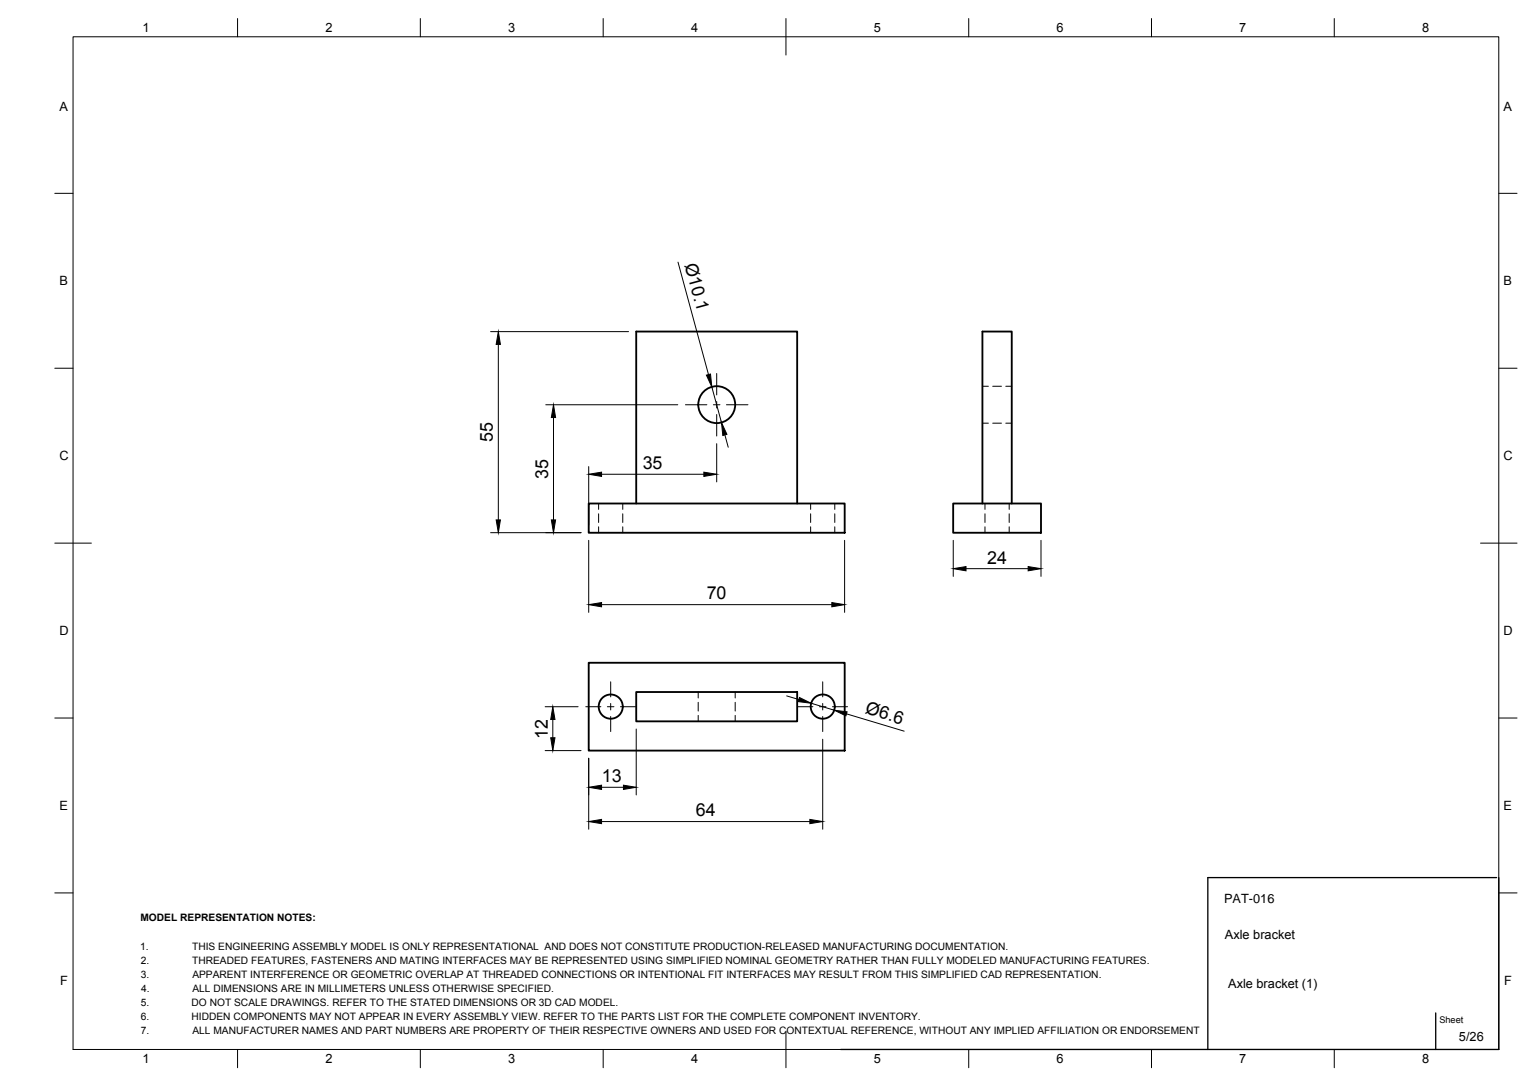
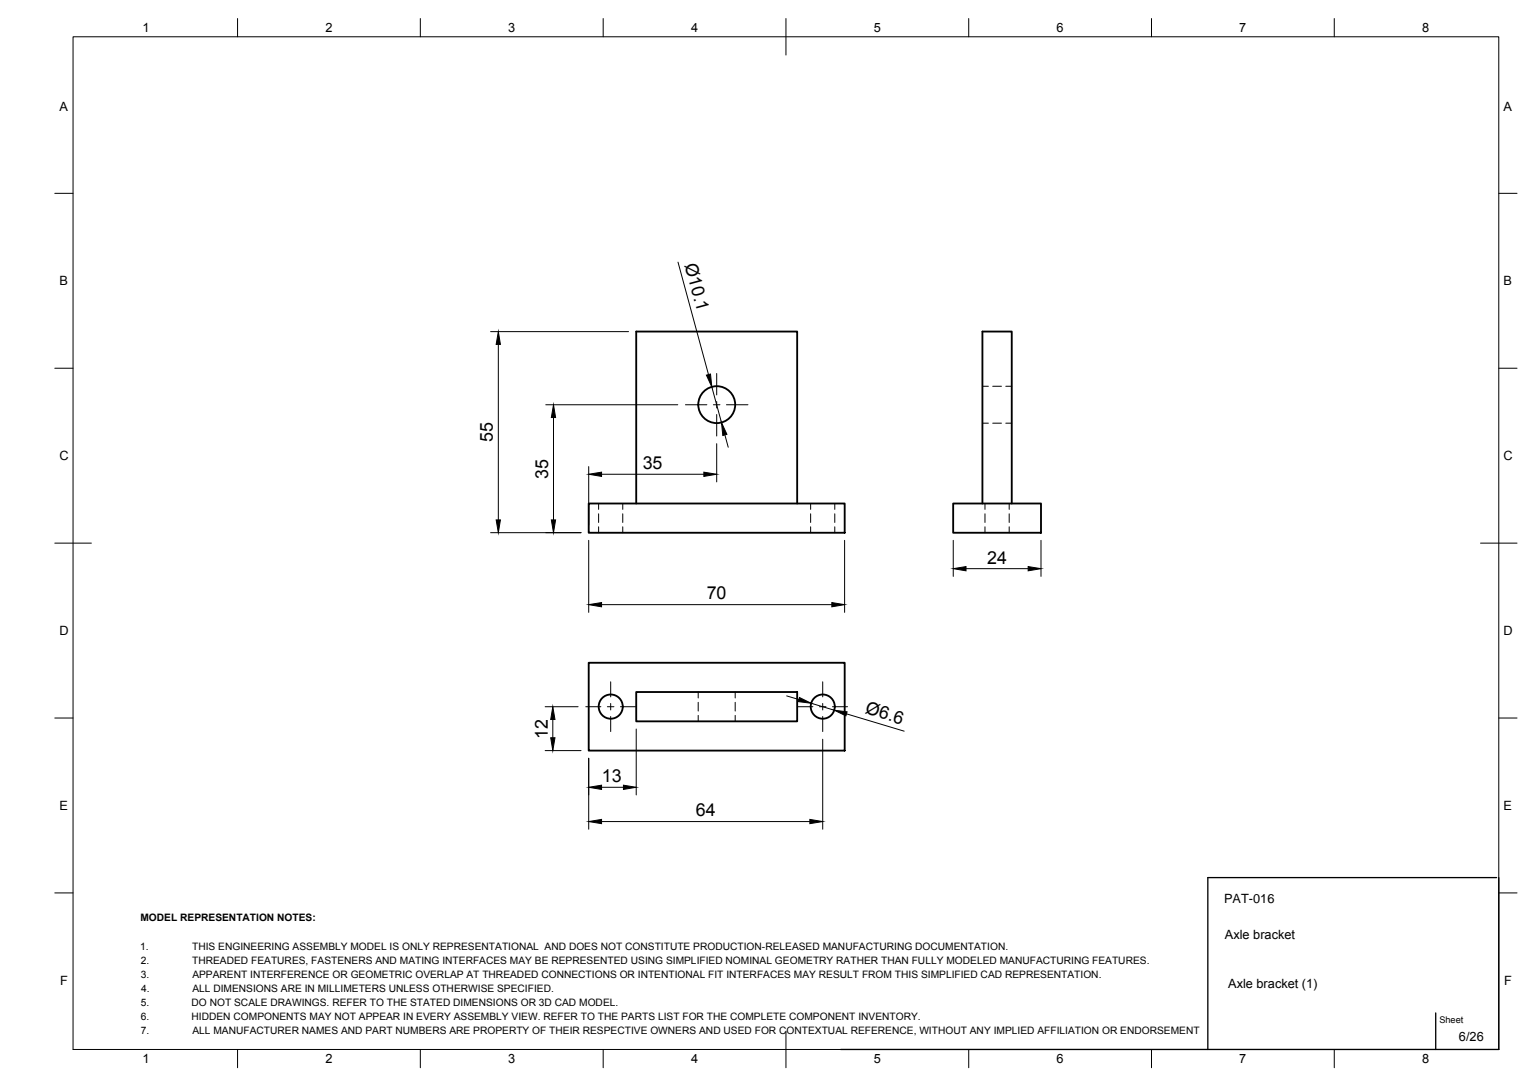
ISO-10303-21;
HEADER;
/* Generated by software containing ST-Developer
 * from STEP Tools, Inc. (www.steptools.com) 
 */

FILE_DESCRIPTION(
/* description */ ('Bracket-mounted idler roller'),
/* implementation_level */ '2;1');

FILE_NAME(
/* name */ 'Axle bracket.step',
/* time_stamp */ '2026-10-28T03:26:42-07:00',
/* author */ (''),
/* organization */ (''),
/* preprocessor_version */ 'ST-DEVELOPER v20.2',
/* originating_system */ 'Autodesk Translation Framework v15.17.0.0',
/* authorisation */ '');

FILE_SCHEMA (('AUTOMOTIVE_DESIGN { 1 0 10303 214 3 1 1 }'));
ENDSEC;

DATA;
#10=MECHANICAL_DESIGN_GEOMETRIC_PRESENTATION_REPRESENTATION('',(#280),#6241);
#238=SHAPE_REPRESENTATION_RELATIONSHIP('SRR','None',#6342,#259);
#259=ADVANCED_BREP_SHAPE_REPRESENTATION('',(#309),#6218);
#280=STYLED_ITEM('',(#6538),#309);
#309=MANIFOLD_SOLID_BREP('Body1',#3182);
#336=FACE_BOUND('',#711,.T.);
#337=FACE_BOUND('',#712,.T.);
#338=FACE_BOUND('',#713,.T.);
#339=FACE_BOUND('',#719,.T.);
#340=FACE_BOUND('',#722,.T.);
#341=FACE_BOUND('',#726,.T.);
#342=FACE_BOUND('',#727,.T.);
#417=PLANE('',#3457);
#418=PLANE('',#3458);
#419=PLANE('',#3459);
#420=PLANE('',#3460);
#421=PLANE('',#3461);
#422=PLANE('',#3462);
#423=PLANE('',#3463);
#424=PLANE('',#3464);
#425=PLANE('',#3465);
#426=PLANE('',#3466);
#427=PLANE('',#3467);
#516=FACE_OUTER_BOUND('',#707,.T.);
#517=FACE_OUTER_BOUND('',#708,.T.);
#518=FACE_OUTER_BOUND('',#709,.T.);
#519=FACE_OUTER_BOUND('',#710,.T.);
#520=FACE_OUTER_BOUND('',#714,.T.);
#521=FACE_OUTER_BOUND('',#715,.T.);
#522=FACE_OUTER_BOUND('',#716,.T.);
#523=FACE_OUTER_BOUND('',#717,.T.);
#524=FACE_OUTER_BOUND('',#718,.T.);
#525=FACE_OUTER_BOUND('',#720,.T.);
#526=FACE_OUTER_BOUND('',#721,.T.);
#527=FACE_OUTER_BOUND('',#723,.T.);
#528=FACE_OUTER_BOUND('',#724,.T.);
#529=FACE_OUTER_BOUND('',#725,.T.);
#707=EDGE_LOOP('',(#2166,#2167,#2168,#2169));
#708=EDGE_LOOP('',(#2170,#2171,#2172,#2173));
#709=EDGE_LOOP('',(#2174,#2175,#2176,#2177));
#710=EDGE_LOOP('',(#2178,#2179,#2180,#2181));
#711=EDGE_LOOP('',(#2182));
#712=EDGE_LOOP('',(#2183));
#713=EDGE_LOOP('',(#2184,#2185,#2186,#2187));
#714=EDGE_LOOP('',(#2188,#2189,#2190,#2191));
#715=EDGE_LOOP('',(#2192,#2193,#2194,#2195));
#716=EDGE_LOOP('',(#2196,#2197,#2198,#2199));
#717=EDGE_LOOP('',(#2200,#2201,#2202,#2203));
#718=EDGE_LOOP('',(#2204,#2205,#2206,#2207));
#719=EDGE_LOOP('',(#2208));
#720=EDGE_LOOP('',(#2209,#2210,#2211,#2212));
#721=EDGE_LOOP('',(#2213,#2214,#2215,#2216));
#722=EDGE_LOOP('',(#2217));
#723=EDGE_LOOP('',(#2218,#2219,#2220,#2221));
#724=EDGE_LOOP('',(#2222,#2223,#2224,#2225));
#725=EDGE_LOOP('',(#2226,#2227,#2228,#2229));
#726=EDGE_LOOP('',(#2230));
#727=EDGE_LOOP('',(#2231));
#979=LINE('',#4957,#1161);
#980=LINE('',#4963,#1162);
#981=LINE('',#4969,#1163);
#982=LINE('',#4974,#1164);
#983=LINE('',#4976,#1165);
#984=LINE('',#4978,#1166);
#985=LINE('',#4979,#1167);
#986=LINE('',#4982,#1168);
#987=LINE('',#4984,#1169);
#988=LINE('',#4986,#1170);
#989=LINE('',#4987,#1171);
#990=LINE('',#4990,#1172);
#991=LINE('',#4992,#1173);
#992=LINE('',#4993,#1174);
#993=LINE('',#4996,#1175);
#994=LINE('',#4998,#1176);
#995=LINE('',#4999,#1177);
#996=LINE('',#5001,#1178);
#997=LINE('',#5003,#1179);
#998=LINE('',#5006,#1180);
#999=LINE('',#5008,#1181);
#1000=LINE('',#5009,#1182);
#1001=LINE('',#5012,#1183);
#1002=LINE('',#5013,#1184);
#1003=LINE('',#5016,#1185);
#1004=LINE('',#5017,#1186);
#1005=LINE('',#5019,#1187);
#1161=VECTOR('',#3896,0.33);
#1162=VECTOR('',#3903,0.33);
#1163=VECTOR('',#3910,0.505);
#1164=VECTOR('',#3915,1.);
#1165=VECTOR('',#3916,1.);
#1166=VECTOR('',#3917,1.);
#1167=VECTOR('',#3918,1.);
#1168=VECTOR('',#3919,1.);
#1169=VECTOR('',#3920,1.);
#1170=VECTOR('',#3921,1.);
#1171=VECTOR('',#3922,1.);
#1172=VECTOR('',#3925,1.);
#1173=VECTOR('',#3926,1.);
#1174=VECTOR('',#3927,1.);
#1175=VECTOR('',#3930,1.);
#1176=VECTOR('',#3931,1.);
#1177=VECTOR('',#3932,1.);
#1178=VECTOR('',#3935,1.);
#1179=VECTOR('',#3938,1.);
#1180=VECTOR('',#3941,1.);
#1181=VECTOR('',#3942,1.);
#1182=VECTOR('',#3943,1.);
#1183=VECTOR('',#3946,1.);
#1184=VECTOR('',#3947,1.);
#1185=VECTOR('',#3950,1.);
#1186=VECTOR('',#3951,1.);
#1187=VECTOR('',#3954,1.);
#1343=CIRCLE('',#3449,0.33);
#1344=CIRCLE('',#3450,0.33);
#1345=CIRCLE('',#3452,0.33);
#1346=CIRCLE('',#3453,0.33);
#1347=CIRCLE('',#3455,0.505);
#1348=CIRCLE('',#3456,0.505);
#1524=VERTEX_POINT('',#4954);
#1525=VERTEX_POINT('',#4956);
#1526=VERTEX_POINT('',#4960);
#1527=VERTEX_POINT('',#4962);
#1528=VERTEX_POINT('',#4966);
#1529=VERTEX_POINT('',#4968);
#1530=VERTEX_POINT('',#4972);
#1531=VERTEX_POINT('',#4973);
#1532=VERTEX_POINT('',#4975);
#1533=VERTEX_POINT('',#4977);
#1534=VERTEX_POINT('',#4980);
#1535=VERTEX_POINT('',#4981);
#1536=VERTEX_POINT('',#4983);
#1537=VERTEX_POINT('',#4985);
#1538=VERTEX_POINT('',#4989);
#1539=VERTEX_POINT('',#4991);
#1540=VERTEX_POINT('',#4995);
#1541=VERTEX_POINT('',#4997);
#1542=VERTEX_POINT('',#5005);
#1543=VERTEX_POINT('',#5007);
#1544=VERTEX_POINT('',#5011);
#1545=VERTEX_POINT('',#5015);
#1785=EDGE_CURVE('',#1524,#1524,#1343,.T.);
#1786=EDGE_CURVE('',#1524,#1525,#979,.T.);
#1787=EDGE_CURVE('',#1525,#1525,#1344,.T.);
#1788=EDGE_CURVE('',#1526,#1526,#1345,.T.);
#1789=EDGE_CURVE('',#1526,#1527,#980,.T.);
#1790=EDGE_CURVE('',#1527,#1527,#1346,.T.);
#1791=EDGE_CURVE('',#1528,#1528,#1347,.T.);
#1792=EDGE_CURVE('',#1528,#1529,#981,.T.);
#1793=EDGE_CURVE('',#1529,#1529,#1348,.T.);
#1794=EDGE_CURVE('',#1530,#1531,#982,.T.);
#1795=EDGE_CURVE('',#1530,#1532,#983,.T.);
#1796=EDGE_CURVE('',#1533,#1532,#984,.T.);
#1797=EDGE_CURVE('',#1531,#1533,#985,.T.);
#1798=EDGE_CURVE('',#1534,#1535,#986,.T.);
#1799=EDGE_CURVE('',#1536,#1534,#987,.T.);
#1800=EDGE_CURVE('',#1537,#1536,#988,.T.);
#1801=EDGE_CURVE('',#1535,#1537,#989,.T.);
#1802=EDGE_CURVE('',#1531,#1538,#990,.T.);
#1803=EDGE_CURVE('',#1539,#1533,#991,.T.);
#1804=EDGE_CURVE('',#1538,#1539,#992,.T.);
#1805=EDGE_CURVE('',#1540,#1530,#993,.T.);
#1806=EDGE_CURVE('',#1540,#1541,#994,.T.);
#1807=EDGE_CURVE('',#1532,#1541,#995,.T.);
#1808=EDGE_CURVE('',#1541,#1539,#996,.T.);
#1809=EDGE_CURVE('',#1538,#1540,#997,.T.);
#1810=EDGE_CURVE('',#1536,#1542,#998,.T.);
#1811=EDGE_CURVE('',#1543,#1542,#999,.T.);
#1812=EDGE_CURVE('',#1537,#1543,#1000,.T.);
#1813=EDGE_CURVE('',#1534,#1544,#1001,.T.);
#1814=EDGE_CURVE('',#1542,#1544,#1002,.T.);
#1815=EDGE_CURVE('',#1535,#1545,#1003,.T.);
#1816=EDGE_CURVE('',#1544,#1545,#1004,.T.);
#1817=EDGE_CURVE('',#1545,#1543,#1005,.T.);
#2166=ORIENTED_EDGE('',*,*,#1785,.F.);
#2167=ORIENTED_EDGE('',*,*,#1786,.T.);
#2168=ORIENTED_EDGE('',*,*,#1787,.F.);
#2169=ORIENTED_EDGE('',*,*,#1786,.F.);
#2170=ORIENTED_EDGE('',*,*,#1788,.F.);
#2171=ORIENTED_EDGE('',*,*,#1789,.T.);
#2172=ORIENTED_EDGE('',*,*,#1790,.F.);
#2173=ORIENTED_EDGE('',*,*,#1789,.F.);
#2174=ORIENTED_EDGE('',*,*,#1791,.F.);
#2175=ORIENTED_EDGE('',*,*,#1792,.T.);
#2176=ORIENTED_EDGE('',*,*,#1793,.F.);
#2177=ORIENTED_EDGE('',*,*,#1792,.F.);
#2178=ORIENTED_EDGE('',*,*,#1794,.F.);
#2179=ORIENTED_EDGE('',*,*,#1795,.T.);
#2180=ORIENTED_EDGE('',*,*,#1796,.F.);
#2181=ORIENTED_EDGE('',*,*,#1797,.F.);
#2182=ORIENTED_EDGE('',*,*,#1787,.T.);
#2183=ORIENTED_EDGE('',*,*,#1790,.T.);
#2184=ORIENTED_EDGE('',*,*,#1798,.F.);
#2185=ORIENTED_EDGE('',*,*,#1799,.F.);
#2186=ORIENTED_EDGE('',*,*,#1800,.F.);
#2187=ORIENTED_EDGE('',*,*,#1801,.F.);
#2188=ORIENTED_EDGE('',*,*,#1802,.F.);
#2189=ORIENTED_EDGE('',*,*,#1797,.T.);
#2190=ORIENTED_EDGE('',*,*,#1803,.F.);
#2191=ORIENTED_EDGE('',*,*,#1804,.F.);
#2192=ORIENTED_EDGE('',*,*,#1805,.F.);
#2193=ORIENTED_EDGE('',*,*,#1806,.T.);
#2194=ORIENTED_EDGE('',*,*,#1807,.F.);
#2195=ORIENTED_EDGE('',*,*,#1795,.F.);
#2196=ORIENTED_EDGE('',*,*,#1796,.T.);
#2197=ORIENTED_EDGE('',*,*,#1807,.T.);
#2198=ORIENTED_EDGE('',*,*,#1808,.T.);
#2199=ORIENTED_EDGE('',*,*,#1803,.T.);
#2200=ORIENTED_EDGE('',*,*,#1794,.T.);
#2201=ORIENTED_EDGE('',*,*,#1802,.T.);
#2202=ORIENTED_EDGE('',*,*,#1809,.T.);
#2203=ORIENTED_EDGE('',*,*,#1805,.T.);
#2204=ORIENTED_EDGE('',*,*,#1800,.T.);
#2205=ORIENTED_EDGE('',*,*,#1810,.T.);
#2206=ORIENTED_EDGE('',*,*,#1811,.F.);
#2207=ORIENTED_EDGE('',*,*,#1812,.F.);
#2208=ORIENTED_EDGE('',*,*,#1791,.T.);
#2209=ORIENTED_EDGE('',*,*,#1799,.T.);
#2210=ORIENTED_EDGE('',*,*,#1813,.T.);
#2211=ORIENTED_EDGE('',*,*,#1814,.F.);
#2212=ORIENTED_EDGE('',*,*,#1810,.F.);
#2213=ORIENTED_EDGE('',*,*,#1798,.T.);
#2214=ORIENTED_EDGE('',*,*,#1815,.T.);
#2215=ORIENTED_EDGE('',*,*,#1816,.F.);
#2216=ORIENTED_EDGE('',*,*,#1813,.F.);
#2217=ORIENTED_EDGE('',*,*,#1793,.T.);
#2218=ORIENTED_EDGE('',*,*,#1801,.T.);
#2219=ORIENTED_EDGE('',*,*,#1812,.T.);
#2220=ORIENTED_EDGE('',*,*,#1817,.F.);
#2221=ORIENTED_EDGE('',*,*,#1815,.F.);
#2222=ORIENTED_EDGE('',*,*,#1817,.T.);
#2223=ORIENTED_EDGE('',*,*,#1811,.T.);
#2224=ORIENTED_EDGE('',*,*,#1814,.T.);
#2225=ORIENTED_EDGE('',*,*,#1816,.T.);
#2226=ORIENTED_EDGE('',*,*,#1809,.F.);
#2227=ORIENTED_EDGE('',*,*,#1804,.T.);
#2228=ORIENTED_EDGE('',*,*,#1808,.F.);
#2229=ORIENTED_EDGE('',*,*,#1806,.F.);
#2230=ORIENTED_EDGE('',*,*,#1785,.T.);
#2231=ORIENTED_EDGE('',*,*,#1788,.T.);
#2928=CYLINDRICAL_SURFACE('',#3448,0.33);
#2929=CYLINDRICAL_SURFACE('',#3451,0.33);
#2930=CYLINDRICAL_SURFACE('',#3454,0.505);
#2991=ADVANCED_FACE('',(#516),#2928,.F.);
#2992=ADVANCED_FACE('',(#517),#2929,.F.);
#2993=ADVANCED_FACE('',(#518),#2930,.F.);
#2994=ADVANCED_FACE('',(#519,#336,#337,#338),#417,.T.);
#2995=ADVANCED_FACE('',(#520),#418,.T.);
#2996=ADVANCED_FACE('',(#521),#419,.T.);
#2997=ADVANCED_FACE('',(#522),#420,.T.);
#2998=ADVANCED_FACE('',(#523),#421,.F.);
#2999=ADVANCED_FACE('',(#524,#339),#422,.T.);
#3000=ADVANCED_FACE('',(#525),#423,.T.);
#3001=ADVANCED_FACE('',(#526,#340),#424,.T.);
#3002=ADVANCED_FACE('',(#527),#425,.T.);
#3003=ADVANCED_FACE('',(#528),#426,.T.);
#3004=ADVANCED_FACE('',(#529,#341,#342),#427,.F.);
#3182=CLOSED_SHELL('',(#2991,#2992,#2993,#2994,#2995,#2996,#2997,#2998,
#2999,#3000,#3001,#3002,#3003,#3004));
#3447=AXIS2_PLACEMENT_3D('',#4952,#3890,#3891);
#3448=AXIS2_PLACEMENT_3D('',#4953,#3892,#3893);
#3449=AXIS2_PLACEMENT_3D('',#4955,#3894,#3895);
#3450=AXIS2_PLACEMENT_3D('',#4958,#3897,#3898);
#3451=AXIS2_PLACEMENT_3D('',#4959,#3899,#3900);
#3452=AXIS2_PLACEMENT_3D('',#4961,#3901,#3902);
#3453=AXIS2_PLACEMENT_3D('',#4964,#3904,#3905);
#3454=AXIS2_PLACEMENT_3D('',#4965,#3906,#3907);
#3455=AXIS2_PLACEMENT_3D('',#4967,#3908,#3909);
#3456=AXIS2_PLACEMENT_3D('',#4970,#3911,#3912);
#3457=AXIS2_PLACEMENT_3D('',#4971,#3913,#3914);
#3458=AXIS2_PLACEMENT_3D('',#4988,#3923,#3924);
#3459=AXIS2_PLACEMENT_3D('',#4994,#3928,#3929);
#3460=AXIS2_PLACEMENT_3D('',#5000,#3933,#3934);
#3461=AXIS2_PLACEMENT_3D('',#5002,#3936,#3937);
#3462=AXIS2_PLACEMENT_3D('',#5004,#3939,#3940);
#3463=AXIS2_PLACEMENT_3D('',#5010,#3944,#3945);
#3464=AXIS2_PLACEMENT_3D('',#5014,#3948,#3949);
#3465=AXIS2_PLACEMENT_3D('',#5018,#3952,#3953);
#3466=AXIS2_PLACEMENT_3D('',#5020,#3955,#3956);
#3467=AXIS2_PLACEMENT_3D('',#5021,#3957,#3958);
#3890=DIRECTION('axis',(0.,0.,1.));
#3891=DIRECTION('refdir',(1.,0.,0.));
#3892=DIRECTION('center_axis',(0.,0.,1.));
#3893=DIRECTION('ref_axis',(1.,0.,0.));
#3894=DIRECTION('center_axis',(0.,0.,1.));
#3895=DIRECTION('ref_axis',(1.,0.,0.));
#3896=DIRECTION('',(0.,0.,1.));
#3897=DIRECTION('center_axis',(0.,0.,-1.));
#3898=DIRECTION('ref_axis',(1.,0.,0.));
#3899=DIRECTION('center_axis',(0.,0.,1.));
#3900=DIRECTION('ref_axis',(1.,0.,0.));
#3901=DIRECTION('center_axis',(0.,0.,1.));
#3902=DIRECTION('ref_axis',(1.,0.,0.));
#3903=DIRECTION('',(0.,0.,1.));
#3904=DIRECTION('center_axis',(0.,0.,-1.));
#3905=DIRECTION('ref_axis',(1.,0.,0.));
#3906=DIRECTION('center_axis',(0.,1.,0.));
#3907=DIRECTION('ref_axis',(1.,0.,0.));
#3908=DIRECTION('center_axis',(0.,1.,0.));
#3909=DIRECTION('ref_axis',(1.,0.,0.));
#3910=DIRECTION('',(0.,1.,0.));
#3911=DIRECTION('center_axis',(0.,-1.,0.));
#3912=DIRECTION('ref_axis',(1.,0.,0.));
#3913=DIRECTION('center_axis',(0.,0.,1.));
#3914=DIRECTION('ref_axis',(1.,0.,0.));
#3915=DIRECTION('',(-1.,0.,0.));
#3916=DIRECTION('',(0.,1.,0.));
#3917=DIRECTION('',(1.,0.,0.));
#3918=DIRECTION('',(0.,1.,0.));
#3919=DIRECTION('',(-1.,0.,0.));
#3920=DIRECTION('',(0.,1.,0.));
#3921=DIRECTION('',(1.,0.,0.));
#3922=DIRECTION('',(0.,-1.,0.));
#3923=DIRECTION('center_axis',(-1.,0.,0.));
#3924=DIRECTION('ref_axis',(0.,0.,1.));
#3925=DIRECTION('',(0.,0.,-1.));
#3926=DIRECTION('',(0.,0.,1.));
#3927=DIRECTION('',(0.,1.,0.));
#3928=DIRECTION('center_axis',(1.,0.,0.));
#3929=DIRECTION('ref_axis',(0.,0.,-1.));
#3930=DIRECTION('',(0.,0.,1.));
#3931=DIRECTION('',(0.,1.,0.));
#3932=DIRECTION('',(0.,0.,-1.));
#3933=DIRECTION('center_axis',(0.,1.,0.));
#3934=DIRECTION('ref_axis',(0.,0.,1.));
#3935=DIRECTION('',(-1.,0.,0.));
#3936=DIRECTION('center_axis',(0.,1.,0.));
#3937=DIRECTION('ref_axis',(1.,0.,0.));
#3938=DIRECTION('',(1.,0.,0.));
#3939=DIRECTION('center_axis',(0.,-1.,0.));
#3940=DIRECTION('ref_axis',(1.,0.,0.));
#3941=DIRECTION('',(0.,0.,1.));
#3942=DIRECTION('',(1.,0.,0.));
#3943=DIRECTION('',(0.,0.,1.));
#3944=DIRECTION('center_axis',(1.,0.,0.));
#3945=DIRECTION('ref_axis',(0.,1.,0.));
#3946=DIRECTION('',(0.,0.,1.));
#3947=DIRECTION('',(0.,1.,0.));
#3948=DIRECTION('center_axis',(0.,1.,0.));
#3949=DIRECTION('ref_axis',(-1.,0.,0.));
#3950=DIRECTION('',(0.,0.,1.));
#3951=DIRECTION('',(-1.,0.,0.));
#3952=DIRECTION('center_axis',(-1.,0.,0.));
#3953=DIRECTION('ref_axis',(0.,-1.,0.));
#3954=DIRECTION('',(0.,-1.,0.));
#3955=DIRECTION('center_axis',(0.,0.,1.));
#3956=DIRECTION('ref_axis',(1.,0.,0.));
#3957=DIRECTION('center_axis',(0.,0.,1.));
#3958=DIRECTION('ref_axis',(1.,0.,0.));
#4952=CARTESIAN_POINT('',(0.,0.,0.));
#4953=CARTESIAN_POINT('Origin',(-2.9,-2.,0.9));
#4954=CARTESIAN_POINT('',(-3.23,-2.,1.));
#4955=CARTESIAN_POINT('Origin',(-2.9,-2.,1.));
#4956=CARTESIAN_POINT('',(-3.23,-2.,1.8));
#4957=CARTESIAN_POINT('',(-3.23,-2.,0.9));
#4958=CARTESIAN_POINT('Origin',(-2.9,-2.,1.8));
#4959=CARTESIAN_POINT('Origin',(2.9,-2.,0.9));
#4960=CARTESIAN_POINT('',(2.57,-2.,1.));
#4961=CARTESIAN_POINT('Origin',(2.9,-2.,1.));
#4962=CARTESIAN_POINT('',(2.57,-2.,1.8));
#4963=CARTESIAN_POINT('',(2.57,-2.,0.9));
#4964=CARTESIAN_POINT('Origin',(2.9,-2.,1.8));
#4965=CARTESIAN_POINT('Origin',(0.,-2.5,4.5));
#4966=CARTESIAN_POINT('',(-0.505,-2.4,4.5));
#4967=CARTESIAN_POINT('Origin',(0.,-2.4,4.5));
#4968=CARTESIAN_POINT('',(-0.505,-1.6,4.5));
#4969=CARTESIAN_POINT('',(-0.505,-2.5,4.5));
#4970=CARTESIAN_POINT('Origin',(0.,-1.6,4.5));
#4971=CARTESIAN_POINT('Origin',(-3.5,-3.2,1.8));
#4972=CARTESIAN_POINT('',(3.5,-3.2,1.8));
#4973=CARTESIAN_POINT('',(-3.5,-3.2,1.8));
#4974=CARTESIAN_POINT('',(3.5,-3.2,1.8));
#4975=CARTESIAN_POINT('',(3.5,-0.8,1.8));
#4976=CARTESIAN_POINT('',(3.5,-3.2,1.8));
#4977=CARTESIAN_POINT('',(-3.5,-0.8,1.8));
#4978=CARTESIAN_POINT('',(3.5,-0.8,1.8));
#4979=CARTESIAN_POINT('',(-3.5,-3.2,1.8));
#4980=CARTESIAN_POINT('',(2.2,-1.6,1.8));
#4981=CARTESIAN_POINT('',(-2.2,-1.6,1.8));
#4982=CARTESIAN_POINT('',(-0.65,-1.6,1.8));
#4983=CARTESIAN_POINT('',(2.2,-2.4,1.8));
#4984=CARTESIAN_POINT('',(2.2,-2.8,1.8));
#4985=CARTESIAN_POINT('',(-2.2,-2.4,1.8));
#4986=CARTESIAN_POINT('',(-2.85,-2.4,1.8));
#4987=CARTESIAN_POINT('',(-2.2,-2.4,1.8));
#4988=CARTESIAN_POINT('Origin',(-3.5,-3.2,1.));
#4989=CARTESIAN_POINT('',(-3.5,-3.2,1.));
#4990=CARTESIAN_POINT('',(-3.5,-3.2,1.8));
#4991=CARTESIAN_POINT('',(-3.5,-0.8,1.));
#4992=CARTESIAN_POINT('',(-3.5,-0.8,1.8));
#4993=CARTESIAN_POINT('',(-3.5,-3.2,1.));
#4994=CARTESIAN_POINT('Origin',(3.5,-3.2,1.8));
#4995=CARTESIAN_POINT('',(3.5,-3.2,1.));
#4996=CARTESIAN_POINT('',(3.5,-3.2,1.));
#4997=CARTESIAN_POINT('',(3.5,-0.8,1.));
#4998=CARTESIAN_POINT('',(3.5,-3.2,1.));
#4999=CARTESIAN_POINT('',(3.5,-0.8,1.));
#5000=CARTESIAN_POINT('Origin',(0.,-0.8,1.4));
#5001=CARTESIAN_POINT('',(-3.5,-0.8,1.));
#5002=CARTESIAN_POINT('Origin',(0.,-3.2,1.4));
#5003=CARTESIAN_POINT('',(-3.5,-3.2,1.));
#5004=CARTESIAN_POINT('Origin',(-2.2,-2.4,1.));
#5005=CARTESIAN_POINT('',(2.2,-2.4,6.5));
#5006=CARTESIAN_POINT('',(2.2,-2.4,1.));
#5007=CARTESIAN_POINT('',(-2.2,-2.4,6.5));
#5008=CARTESIAN_POINT('',(-2.2,-2.4,6.5));
#5009=CARTESIAN_POINT('',(-2.2,-2.4,1.));
#5010=CARTESIAN_POINT('Origin',(2.2,-2.4,1.));
#5011=CARTESIAN_POINT('',(2.2,-1.6,6.5));
#5012=CARTESIAN_POINT('',(2.2,-1.6,1.));
#5013=CARTESIAN_POINT('',(2.2,-2.4,6.5));
#5014=CARTESIAN_POINT('Origin',(2.2,-1.6,1.));
#5015=CARTESIAN_POINT('',(-2.2,-1.6,6.5));
#5016=CARTESIAN_POINT('',(-2.2,-1.6,1.));
#5017=CARTESIAN_POINT('',(2.2,-1.6,6.5));
#5018=CARTESIAN_POINT('Origin',(-2.2,-1.6,1.));
#5019=CARTESIAN_POINT('',(-2.2,-1.6,6.5));
#5020=CARTESIAN_POINT('Origin',(0.,-2.,6.5));
#5021=CARTESIAN_POINT('Origin',(0.,-2.,1.));
#6192=UNCERTAINTY_MEASURE_WITH_UNIT(LENGTH_MEASURE(0.001),#6242,
'DISTANCE_ACCURACY_VALUE',
'Maximum model space distance between geometric entities at asserted c
onnectivities');
#6215=UNCERTAINTY_MEASURE_WITH_UNIT(LENGTH_MEASURE(0.001),#6242,
'DISTANCE_ACCURACY_VALUE',
'Maximum model space distance between geometric entities at asserted c
onnectivities');
#6218=(
GEOMETRIC_REPRESENTATION_CONTEXT(3)
GLOBAL_UNCERTAINTY_ASSIGNED_CONTEXT((#6192))
GLOBAL_UNIT_ASSIGNED_CONTEXT((#6242,#6244,#6245))
REPRESENTATION_CONTEXT('','3D')
);
#6241=(
GEOMETRIC_REPRESENTATION_CONTEXT(3)
GLOBAL_UNCERTAINTY_ASSIGNED_CONTEXT((#6215))
GLOBAL_UNIT_ASSIGNED_CONTEXT((#6242,#6244,#6245))
REPRESENTATION_CONTEXT('','3D')
);
#6242=(
LENGTH_UNIT()
NAMED_UNIT(*)
SI_UNIT(.CENTI.,.METRE.)
);
#6244=(
NAMED_UNIT(*)
PLANE_ANGLE_UNIT()
SI_UNIT($,.RADIAN.)
);
#6245=(
NAMED_UNIT(*)
SI_UNIT($,.STERADIAN.)
SOLID_ANGLE_UNIT()
);
#6248=SHAPE_DEFINITION_REPRESENTATION(#6273,#6342);
#6273=PRODUCT_DEFINITION_SHAPE('',$,#6368);
#6342=SHAPE_REPRESENTATION('',(#3447),#6218);
#6365=PRODUCT_DEFINITION_CONTEXT('part definition',#6442,'design');
#6368=PRODUCT_DEFINITION('Axle bracket','Axle bracket',#6393,#6365);
#6393=PRODUCT_DEFINITION_FORMATION('',$,#6446);
#6442=APPLICATION_CONTEXT(
'Core Data for Automotive Mechanical Design Process');
#6443=PRODUCT_CONTEXT('part definition',#6442,'mechanical');
#6446=PRODUCT('Axle bracket','Axle bracket','Axle bracket',(#6443));
#6532=COLOUR_RGB('Grey',0.48,0.52,0.57);
#6533=FILL_AREA_STYLE_COLOUR('',#6532);
#6534=FILL_AREA_STYLE('',(#6533));
#6535=SURFACE_STYLE_FILL_AREA(#6534);
#6536=SURFACE_SIDE_STYLE('',(#6535));
#6537=SURFACE_STYLE_USAGE(.BOTH.,#6536);
#6538=PRESENTATION_STYLE_ASSIGNMENT((#6537));
ENDSEC;
END-ISO-10303-21;
